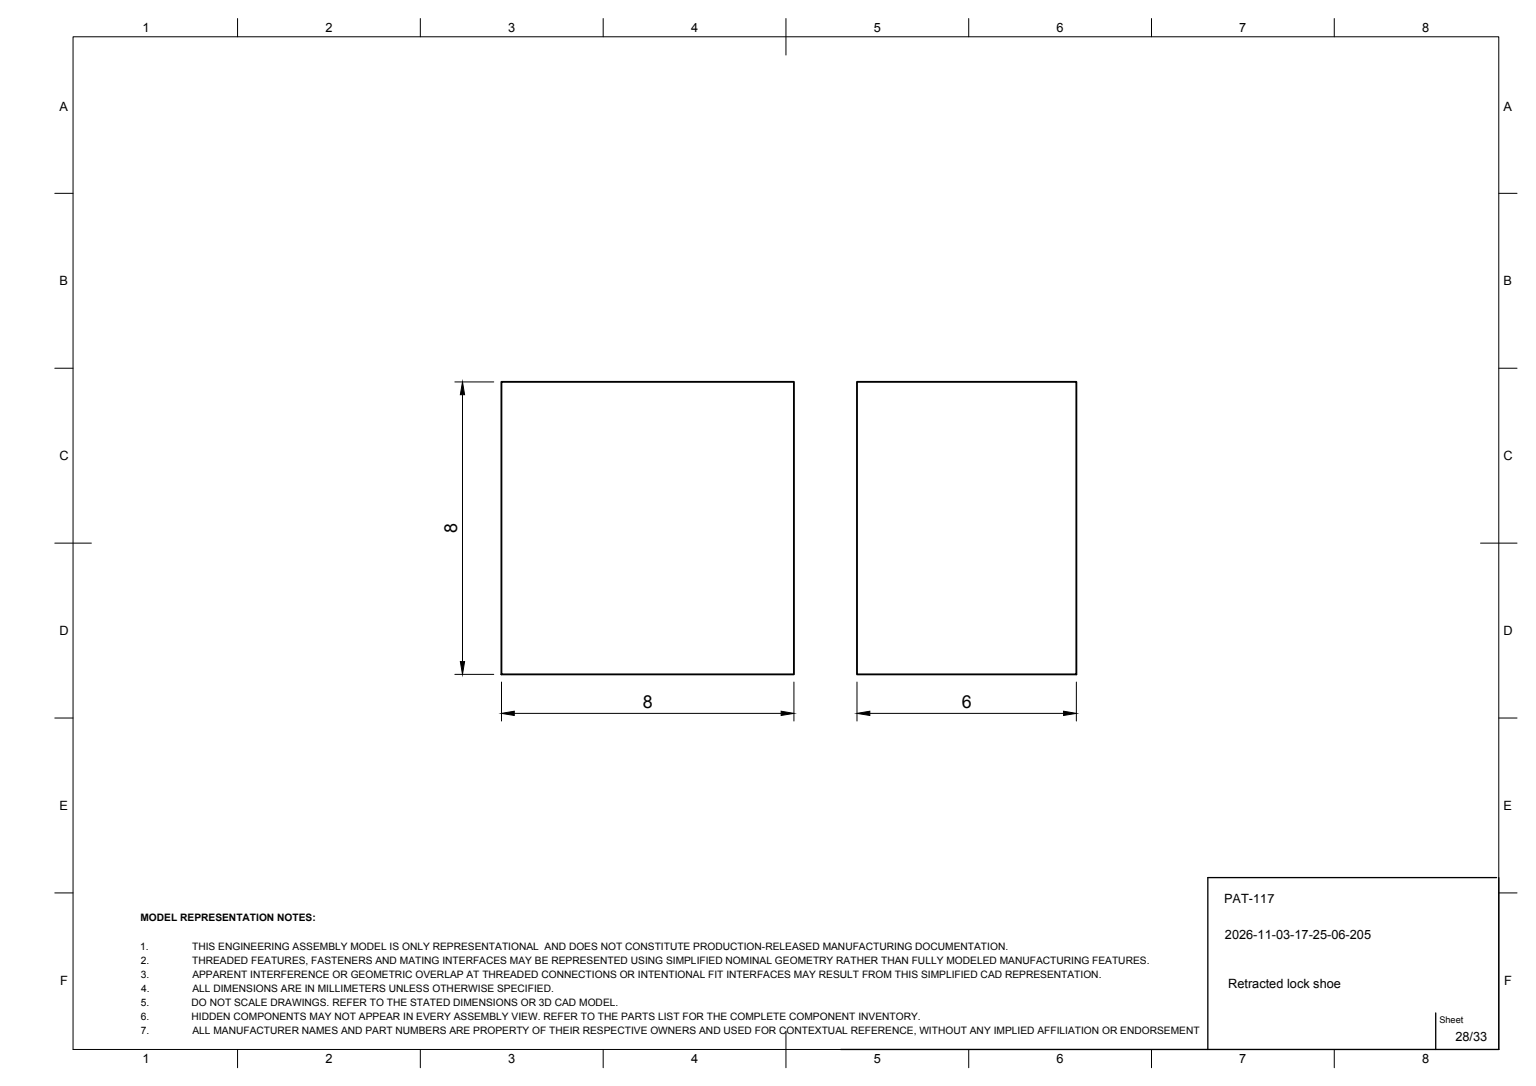
ISO-10303-21;
HEADER;
/* Generated by software containing ST-Developer
 * from STEP Tools, Inc. (www.steptools.com) 
 */

FILE_DESCRIPTION(
/* description */ ('Counterbalanced vertical column'),
/* implementation_level */ '2;1');

FILE_NAME(
/* name */ 'Retracted lock shoe.step',
/* time_stamp */ '2026-10-29T16:47:22-07:00',
/* author */ (''),
/* organization */ (''),
/* preprocessor_version */ 'ST-DEVELOPER v20.2',
/* originating_system */ 'Autodesk Translation Framework v15.17.0.0',
/* authorisation */ '');

FILE_SCHEMA (('AUTOMOTIVE_DESIGN { 1 0 10303 214 3 1 1 }'));
ENDSEC;

DATA;
#10=MECHANICAL_DESIGN_GEOMETRIC_PRESENTATION_REPRESENTATION('',(#378),#15040);
#308=SHAPE_REPRESENTATION_RELATIONSHIP('SRR','None',#15213,#343);
#343=ADVANCED_BREP_SHAPE_REPRESENTATION('',(#411),#15032);
#378=STYLED_ITEM('',(#15450),#411);
#411=MANIFOLD_SOLID_BREP('Body1',#7103);
#757=PLANE('',#8034);
#758=PLANE('',#8035);
#759=PLANE('',#8036);
#760=PLANE('',#8037);
#761=PLANE('',#8038);
#762=PLANE('',#8039);
#1145=FACE_OUTER_BOUND('',#1658,.T.);
#1146=FACE_OUTER_BOUND('',#1659,.T.);
#1147=FACE_OUTER_BOUND('',#1660,.T.);
#1148=FACE_OUTER_BOUND('',#1661,.T.);
#1149=FACE_OUTER_BOUND('',#1662,.T.);
#1150=FACE_OUTER_BOUND('',#1663,.T.);
#1658=EDGE_LOOP('',(#6174,#6175,#6176,#6177));
#1659=EDGE_LOOP('',(#6178,#6179,#6180,#6181));
#1660=EDGE_LOOP('',(#6182,#6183,#6184,#6185));
#1661=EDGE_LOOP('',(#6186,#6187,#6188,#6189));
#1662=EDGE_LOOP('',(#6190,#6191,#6192,#6193));
#1663=EDGE_LOOP('',(#6194,#6195,#6196,#6197));
#2257=LINE('',#14481,#2928);
#2258=LINE('',#14483,#2929);
#2259=LINE('',#14485,#2930);
#2260=LINE('',#14486,#2931);
#2261=LINE('',#14489,#2932);
#2262=LINE('',#14491,#2933);
#2263=LINE('',#14492,#2934);
#2264=LINE('',#14495,#2935);
#2265=LINE('',#14497,#2936);
#2266=LINE('',#14498,#2937);
#2267=LINE('',#14500,#2938);
#2268=LINE('',#14501,#2939);
#2928=VECTOR('',#9801,1.);
#2929=VECTOR('',#9802,1.);
#2930=VECTOR('',#9803,1.);
#2931=VECTOR('',#9804,1.);
#2932=VECTOR('',#9807,1.);
#2933=VECTOR('',#9808,1.);
#2934=VECTOR('',#9809,1.);
#2935=VECTOR('',#9812,1.);
#2936=VECTOR('',#9813,1.);
#2937=VECTOR('',#9814,1.);
#2938=VECTOR('',#9817,1.);
#2939=VECTOR('',#9818,1.);
#3764=VERTEX_POINT('',#14479);
#3765=VERTEX_POINT('',#14480);
#3766=VERTEX_POINT('',#14482);
#3767=VERTEX_POINT('',#14484);
#3768=VERTEX_POINT('',#14488);
#3769=VERTEX_POINT('',#14490);
#3770=VERTEX_POINT('',#14494);
#3771=VERTEX_POINT('',#14496);
#4588=EDGE_CURVE('',#3764,#3765,#2257,.T.);
#4589=EDGE_CURVE('',#3765,#3766,#2258,.T.);
#4590=EDGE_CURVE('',#3767,#3766,#2259,.T.);
#4591=EDGE_CURVE('',#3764,#3767,#2260,.T.);
#4592=EDGE_CURVE('',#3768,#3764,#2261,.T.);
#4593=EDGE_CURVE('',#3769,#3767,#2262,.T.);
#4594=EDGE_CURVE('',#3768,#3769,#2263,.T.);
#4595=EDGE_CURVE('',#3770,#3768,#2264,.T.);
#4596=EDGE_CURVE('',#3771,#3769,#2265,.T.);
#4597=EDGE_CURVE('',#3770,#3771,#2266,.T.);
#4598=EDGE_CURVE('',#3765,#3770,#2267,.T.);
#4599=EDGE_CURVE('',#3766,#3771,#2268,.T.);
#6174=ORIENTED_EDGE('',*,*,#4588,.T.);
#6175=ORIENTED_EDGE('',*,*,#4589,.T.);
#6176=ORIENTED_EDGE('',*,*,#4590,.F.);
#6177=ORIENTED_EDGE('',*,*,#4591,.F.);
#6178=ORIENTED_EDGE('',*,*,#4592,.T.);
#6179=ORIENTED_EDGE('',*,*,#4591,.T.);
#6180=ORIENTED_EDGE('',*,*,#4593,.F.);
#6181=ORIENTED_EDGE('',*,*,#4594,.F.);
#6182=ORIENTED_EDGE('',*,*,#4595,.T.);
#6183=ORIENTED_EDGE('',*,*,#4594,.T.);
#6184=ORIENTED_EDGE('',*,*,#4596,.F.);
#6185=ORIENTED_EDGE('',*,*,#4597,.F.);
#6186=ORIENTED_EDGE('',*,*,#4598,.T.);
#6187=ORIENTED_EDGE('',*,*,#4597,.T.);
#6188=ORIENTED_EDGE('',*,*,#4599,.F.);
#6189=ORIENTED_EDGE('',*,*,#4589,.F.);
#6190=ORIENTED_EDGE('',*,*,#4599,.T.);
#6191=ORIENTED_EDGE('',*,*,#4596,.T.);
#6192=ORIENTED_EDGE('',*,*,#4593,.T.);
#6193=ORIENTED_EDGE('',*,*,#4590,.T.);
#6194=ORIENTED_EDGE('',*,*,#4598,.F.);
#6195=ORIENTED_EDGE('',*,*,#4588,.F.);
#6196=ORIENTED_EDGE('',*,*,#4592,.F.);
#6197=ORIENTED_EDGE('',*,*,#4595,.F.);
#6987=ADVANCED_FACE('',(#1145),#757,.T.);
#6988=ADVANCED_FACE('',(#1146),#758,.T.);
#6989=ADVANCED_FACE('',(#1147),#759,.T.);
#6990=ADVANCED_FACE('',(#1148),#760,.T.);
#6991=ADVANCED_FACE('',(#1149),#761,.T.);
#6992=ADVANCED_FACE('',(#1150),#762,.F.);
#7103=CLOSED_SHELL('',(#6987,#6988,#6989,#6990,#6991,#6992));
#8033=AXIS2_PLACEMENT_3D('',#14477,#9797,#9798);
#8034=AXIS2_PLACEMENT_3D('',#14478,#9799,#9800);
#8035=AXIS2_PLACEMENT_3D('',#14487,#9805,#9806);
#8036=AXIS2_PLACEMENT_3D('',#14493,#9810,#9811);
#8037=AXIS2_PLACEMENT_3D('',#14499,#9815,#9816);
#8038=AXIS2_PLACEMENT_3D('',#14502,#9819,#9820);
#8039=AXIS2_PLACEMENT_3D('',#14503,#9821,#9822);
#9797=DIRECTION('axis',(0.,0.,1.));
#9798=DIRECTION('refdir',(1.,0.,0.));
#9799=DIRECTION('center_axis',(0.,1.,0.));
#9800=DIRECTION('ref_axis',(-1.,0.,0.));
#9801=DIRECTION('',(-1.,0.,0.));
#9802=DIRECTION('',(0.,0.,1.));
#9803=DIRECTION('',(-1.,0.,0.));
#9804=DIRECTION('',(0.,0.,1.));
#9805=DIRECTION('center_axis',(1.,0.,0.));
#9806=DIRECTION('ref_axis',(0.,1.,0.));
#9807=DIRECTION('',(0.,1.,0.));
#9808=DIRECTION('',(0.,1.,0.));
#9809=DIRECTION('',(0.,0.,1.));
#9810=DIRECTION('center_axis',(0.,-1.,0.));
#9811=DIRECTION('ref_axis',(1.,0.,0.));
#9812=DIRECTION('',(1.,0.,0.));
#9813=DIRECTION('',(1.,0.,0.));
#9814=DIRECTION('',(0.,0.,1.));
#9815=DIRECTION('center_axis',(-1.,0.,0.));
#9816=DIRECTION('ref_axis',(0.,-1.,0.));
#9817=DIRECTION('',(0.,-1.,0.));
#9818=DIRECTION('',(0.,-1.,0.));
#9819=DIRECTION('center_axis',(0.,0.,1.));
#9820=DIRECTION('ref_axis',(1.,0.,0.));
#9821=DIRECTION('center_axis',(0.,0.,1.));
#9822=DIRECTION('ref_axis',(1.,0.,0.));
#14477=CARTESIAN_POINT('',(0.,0.,0.));
#14478=CARTESIAN_POINT('Origin',(2.2,1.8,17.2));
#14479=CARTESIAN_POINT('',(2.2,1.8,17.2));
#14480=CARTESIAN_POINT('',(1.4,1.8,17.2));
#14481=CARTESIAN_POINT('',(2.2,1.8,17.2));
#14482=CARTESIAN_POINT('',(1.4,1.8,18.));
#14483=CARTESIAN_POINT('',(1.4,1.8,17.2));
#14484=CARTESIAN_POINT('',(2.2,1.8,18.));
#14485=CARTESIAN_POINT('',(2.2,1.8,18.));
#14486=CARTESIAN_POINT('',(2.2,1.8,17.2));
#14487=CARTESIAN_POINT('Origin',(2.2,1.2,17.2));
#14488=CARTESIAN_POINT('',(2.2,1.2,17.2));
#14489=CARTESIAN_POINT('',(2.2,1.2,17.2));
#14490=CARTESIAN_POINT('',(2.2,1.2,18.));
#14491=CARTESIAN_POINT('',(2.2,1.2,18.));
#14492=CARTESIAN_POINT('',(2.2,1.2,17.2));
#14493=CARTESIAN_POINT('Origin',(1.4,1.2,17.2));
#14494=CARTESIAN_POINT('',(1.4,1.2,17.2));
#14495=CARTESIAN_POINT('',(1.4,1.2,17.2));
#14496=CARTESIAN_POINT('',(1.4,1.2,18.));
#14497=CARTESIAN_POINT('',(1.4,1.2,18.));
#14498=CARTESIAN_POINT('',(1.4,1.2,17.2));
#14499=CARTESIAN_POINT('Origin',(1.4,1.8,17.2));
#14500=CARTESIAN_POINT('',(1.4,1.8,17.2));
#14501=CARTESIAN_POINT('',(1.4,1.8,18.));
#14502=CARTESIAN_POINT('Origin',(1.8,1.5,18.));
#14503=CARTESIAN_POINT('Origin',(1.8,1.5,17.2));
#14992=UNCERTAINTY_MEASURE_WITH_UNIT(LENGTH_MEASURE(0.001),#15041,
'DISTANCE_ACCURACY_VALUE',
'Maximum model space distance between geometric entities at asserted c
onnectivities');
#15000=UNCERTAINTY_MEASURE_WITH_UNIT(LENGTH_MEASURE(0.001),#15041,
'DISTANCE_ACCURACY_VALUE',
'Maximum model space distance between geometric entities at asserted c
onnectivities');
#15032=(
GEOMETRIC_REPRESENTATION_CONTEXT(3)
GLOBAL_UNCERTAINTY_ASSIGNED_CONTEXT((#14992))
GLOBAL_UNIT_ASSIGNED_CONTEXT((#15041,#15043,#15044))
REPRESENTATION_CONTEXT('','3D')
);
#15040=(
GEOMETRIC_REPRESENTATION_CONTEXT(3)
GLOBAL_UNCERTAINTY_ASSIGNED_CONTEXT((#15000))
GLOBAL_UNIT_ASSIGNED_CONTEXT((#15041,#15043,#15044))
REPRESENTATION_CONTEXT('','3D')
);
#15041=(
LENGTH_UNIT()
NAMED_UNIT(*)
SI_UNIT(.CENTI.,.METRE.)
);
#15043=(
NAMED_UNIT(*)
PLANE_ANGLE_UNIT()
SI_UNIT($,.RADIAN.)
);
#15044=(
NAMED_UNIT(*)
SI_UNIT($,.STERADIAN.)
SOLID_ANGLE_UNIT()
);
#15076=SHAPE_DEFINITION_REPRESENTATION(#15115,#15213);
#15115=PRODUCT_DEFINITION_SHAPE('',$,#15253);
#15213=SHAPE_REPRESENTATION('',(#8033),#15032);
#15221=PRODUCT_DEFINITION_CONTEXT('part definition',#15340,'design');
#15253=PRODUCT_DEFINITION('Retracted lock shoe','Retracted lock shoe',#15292,
#15221);
#15292=PRODUCT_DEFINITION_FORMATION('',$,#15373);
#15340=APPLICATION_CONTEXT(
'Core Data for Automotive Mechanical Design Process');
#15341=PRODUCT_CONTEXT('part definition',#15340,'mechanical');
#15373=PRODUCT('Retracted lock shoe','Retracted lock shoe',
'Retracted lock shoe',(#15341));
#15444=COLOUR_RGB('Sky Blue',0.24,0.69,0.87);
#15445=FILL_AREA_STYLE_COLOUR('',#15444);
#15446=FILL_AREA_STYLE('',(#15445));
#15447=SURFACE_STYLE_FILL_AREA(#15446);
#15448=SURFACE_SIDE_STYLE('',(#15447));
#15449=SURFACE_STYLE_USAGE(.BOTH.,#15448);
#15450=PRESENTATION_STYLE_ASSIGNMENT((#15449));
ENDSEC;
END-ISO-10303-21;
